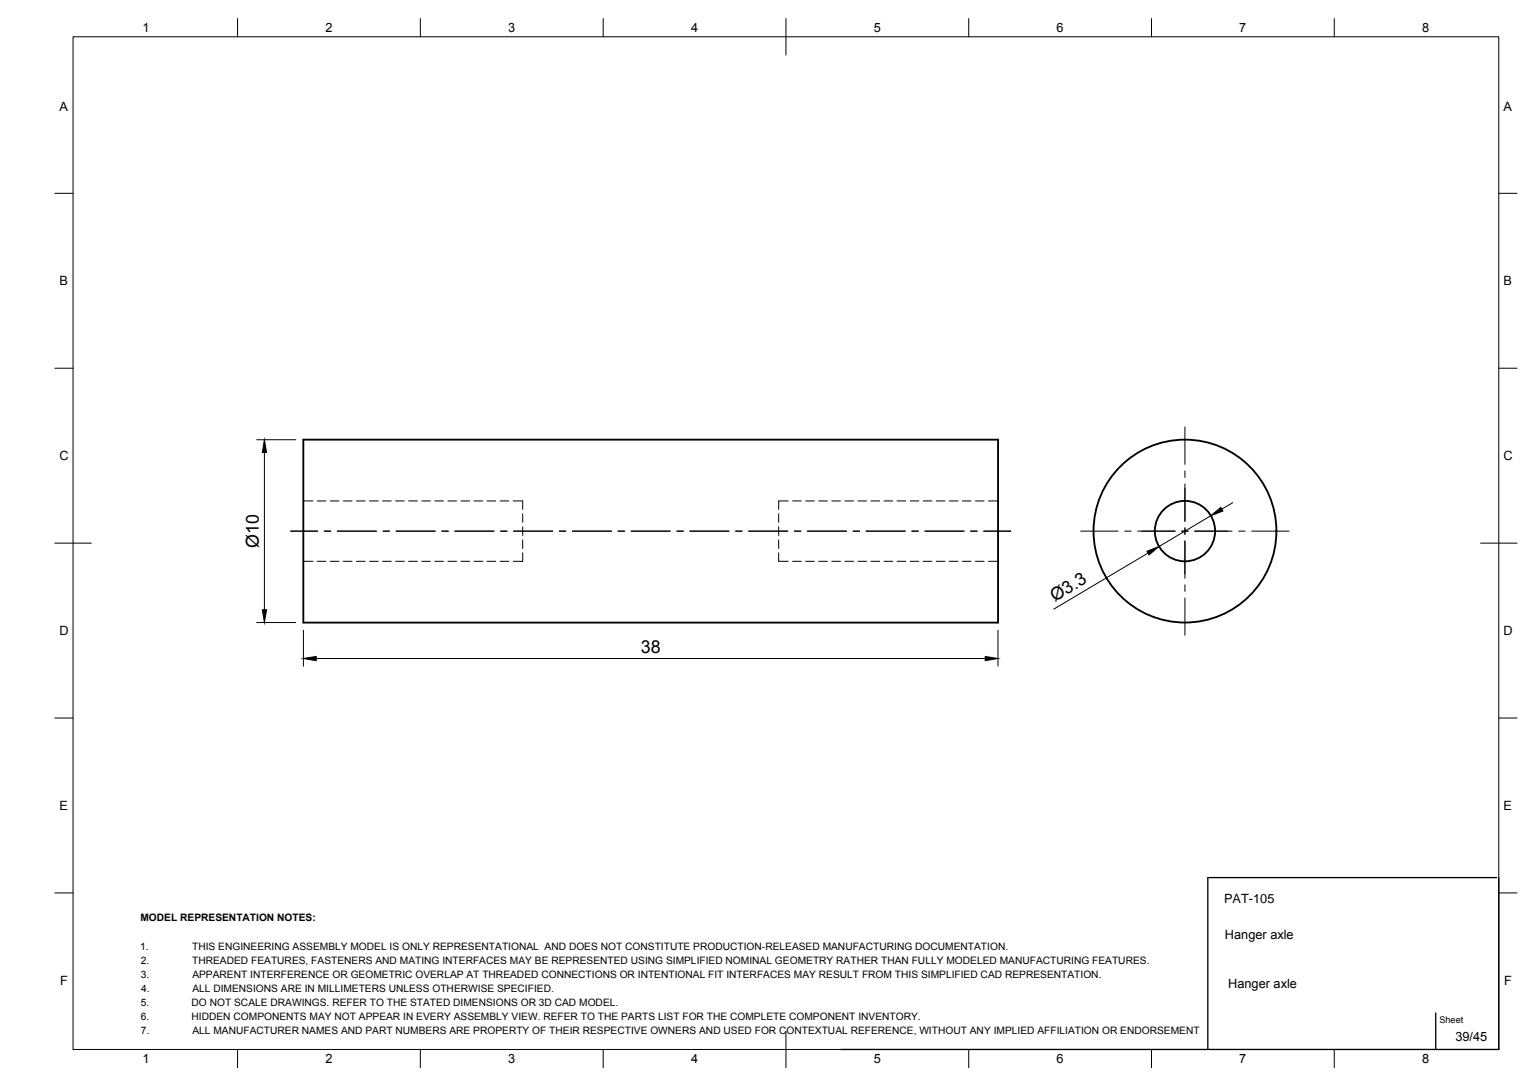
ISO-10303-21;
HEADER;
/* Generated by software containing ST-Developer
 * from STEP Tools, Inc. (www.steptools.com) 
 */

FILE_DESCRIPTION(
/* description */ ('Torque wrench calibration arm'),
/* implementation_level */ '2;1');

FILE_NAME(
/* name */ 'Hanger axle.step',
/* time_stamp */ '2026-10-28T03:24:52-07:00',
/* author */ (''),
/* organization */ (''),
/* preprocessor_version */ 'ST-DEVELOPER v20.2',
/* originating_system */ 'Autodesk Translation Framework v15.17.0.0',
/* authorisation */ '');

FILE_SCHEMA (('AUTOMOTIVE_DESIGN { 1 0 10303 214 3 1 1 }'));
ENDSEC;

DATA;
#10=MECHANICAL_DESIGN_GEOMETRIC_PRESENTATION_REPRESENTATION('',(#472),#12783);
#381=SHAPE_REPRESENTATION_RELATIONSHIP('SRR','None',#12966,#418);
#418=ADVANCED_BREP_SHAPE_REPRESENTATION('',(#524),#12775);
#472=STYLED_ITEM('',(#13212),#524);
#524=MANIFOLD_SOLID_BREP('Body1',#6543);
#637=FACE_BOUND('',#1730,.T.);
#638=FACE_BOUND('',#1732,.T.);
#848=PLANE('',#7709);
#849=PLANE('',#7713);
#850=PLANE('',#7717);
#851=PLANE('',#7718);
#1223=FACE_OUTER_BOUND('',#1724,.T.);
#1224=FACE_OUTER_BOUND('',#1725,.T.);
#1225=FACE_OUTER_BOUND('',#1726,.T.);
#1226=FACE_OUTER_BOUND('',#1727,.T.);
#1227=FACE_OUTER_BOUND('',#1728,.T.);
#1228=FACE_OUTER_BOUND('',#1729,.T.);
#1229=FACE_OUTER_BOUND('',#1731,.T.);
#1724=EDGE_LOOP('',(#5837,#5838,#5839,#5840));
#1725=EDGE_LOOP('',(#5841));
#1726=EDGE_LOOP('',(#5842,#5843,#5844,#5845));
#1727=EDGE_LOOP('',(#5846));
#1728=EDGE_LOOP('',(#5847,#5848,#5849,#5850));
#1729=EDGE_LOOP('',(#5851));
#1730=EDGE_LOOP('',(#5852));
#1731=EDGE_LOOP('',(#5853));
#1732=EDGE_LOOP('',(#5854));
#2163=LINE('',#12509,#2578);
#2164=LINE('',#12516,#2579);
#2165=LINE('',#12523,#2580);
#2578=VECTOR('',#9683,0.164999999999999);
#2579=VECTOR('',#9692,0.164999999999999);
#2580=VECTOR('',#9701,0.5);
#2934=CIRCLE('',#7707,0.164999999999999);
#2935=CIRCLE('',#7708,0.164999999999999);
#2936=CIRCLE('',#7711,0.164999999999999);
#2937=CIRCLE('',#7712,0.164999999999999);
#2938=CIRCLE('',#7715,0.5);
#2939=CIRCLE('',#7716,0.5);
#3484=VERTEX_POINT('',#12506);
#3485=VERTEX_POINT('',#12508);
#3486=VERTEX_POINT('',#12513);
#3487=VERTEX_POINT('',#12515);
#3488=VERTEX_POINT('',#12520);
#3489=VERTEX_POINT('',#12522);
#4276=EDGE_CURVE('',#3484,#3484,#2934,.T.);
#4277=EDGE_CURVE('',#3484,#3485,#2163,.T.);
#4278=EDGE_CURVE('',#3485,#3485,#2935,.T.);
#4279=EDGE_CURVE('',#3486,#3486,#2936,.T.);
#4280=EDGE_CURVE('',#3486,#3487,#2164,.T.);
#4281=EDGE_CURVE('',#3487,#3487,#2937,.T.);
#4282=EDGE_CURVE('',#3488,#3488,#2938,.T.);
#4283=EDGE_CURVE('',#3488,#3489,#2165,.T.);
#4284=EDGE_CURVE('',#3489,#3489,#2939,.T.);
#5837=ORIENTED_EDGE('',*,*,#4276,.F.);
#5838=ORIENTED_EDGE('',*,*,#4277,.T.);
#5839=ORIENTED_EDGE('',*,*,#4278,.F.);
#5840=ORIENTED_EDGE('',*,*,#4277,.F.);
#5841=ORIENTED_EDGE('',*,*,#4276,.T.);
#5842=ORIENTED_EDGE('',*,*,#4279,.F.);
#5843=ORIENTED_EDGE('',*,*,#4280,.T.);
#5844=ORIENTED_EDGE('',*,*,#4281,.T.);
#5845=ORIENTED_EDGE('',*,*,#4280,.F.);
#5846=ORIENTED_EDGE('',*,*,#4281,.F.);
#5847=ORIENTED_EDGE('',*,*,#4282,.F.);
#5848=ORIENTED_EDGE('',*,*,#4283,.T.);
#5849=ORIENTED_EDGE('',*,*,#4284,.T.);
#5850=ORIENTED_EDGE('',*,*,#4283,.F.);
#5851=ORIENTED_EDGE('',*,*,#4282,.T.);
#5852=ORIENTED_EDGE('',*,*,#4278,.T.);
#5853=ORIENTED_EDGE('',*,*,#4284,.F.);
#5854=ORIENTED_EDGE('',*,*,#4279,.T.);
#6083=CYLINDRICAL_SURFACE('',#7706,0.164999999999999);
#6084=CYLINDRICAL_SURFACE('',#7710,0.164999999999999);
#6085=CYLINDRICAL_SURFACE('',#7714,0.5);
#6448=ADVANCED_FACE('',(#1223),#6083,.F.);
#6449=ADVANCED_FACE('',(#1224),#848,.T.);
#6450=ADVANCED_FACE('',(#1225),#6084,.F.);
#6451=ADVANCED_FACE('',(#1226),#849,.F.);
#6452=ADVANCED_FACE('',(#1227),#6085,.T.);
#6453=ADVANCED_FACE('',(#1228,#637),#850,.T.);
#6454=ADVANCED_FACE('',(#1229,#638),#851,.F.);
#6543=CLOSED_SHELL('',(#6448,#6449,#6450,#6451,#6452,#6453,#6454));
#7705=AXIS2_PLACEMENT_3D('',#12504,#9677,#9678);
#7706=AXIS2_PLACEMENT_3D('',#12505,#9679,#9680);
#7707=AXIS2_PLACEMENT_3D('',#12507,#9681,#9682);
#7708=AXIS2_PLACEMENT_3D('',#12510,#9684,#9685);
#7709=AXIS2_PLACEMENT_3D('',#12511,#9686,#9687);
#7710=AXIS2_PLACEMENT_3D('',#12512,#9688,#9689);
#7711=AXIS2_PLACEMENT_3D('',#12514,#9690,#9691);
#7712=AXIS2_PLACEMENT_3D('',#12517,#9693,#9694);
#7713=AXIS2_PLACEMENT_3D('',#12518,#9695,#9696);
#7714=AXIS2_PLACEMENT_3D('',#12519,#9697,#9698);
#7715=AXIS2_PLACEMENT_3D('',#12521,#9699,#9700);
#7716=AXIS2_PLACEMENT_3D('',#12524,#9702,#9703);
#7717=AXIS2_PLACEMENT_3D('',#12525,#9704,#9705);
#7718=AXIS2_PLACEMENT_3D('',#12526,#9706,#9707);
#9677=DIRECTION('axis',(0.,0.,1.));
#9678=DIRECTION('refdir',(1.,0.,0.));
#9679=DIRECTION('center_axis',(0.,1.,0.));
#9680=DIRECTION('ref_axis',(1.,0.,0.));
#9681=DIRECTION('center_axis',(0.,1.,0.));
#9682=DIRECTION('ref_axis',(1.,0.,0.));
#9683=DIRECTION('',(0.,1.,0.));
#9684=DIRECTION('center_axis',(0.,-1.,0.));
#9685=DIRECTION('ref_axis',(1.,0.,0.));
#9686=DIRECTION('center_axis',(0.,1.,0.));
#9687=DIRECTION('ref_axis',(1.,0.,0.));
#9688=DIRECTION('center_axis',(0.,1.,0.));
#9689=DIRECTION('ref_axis',(1.,0.,0.));
#9690=DIRECTION('center_axis',(0.,1.,0.));
#9691=DIRECTION('ref_axis',(1.,0.,0.));
#9692=DIRECTION('',(0.,1.,0.));
#9693=DIRECTION('center_axis',(0.,1.,0.));
#9694=DIRECTION('ref_axis',(1.,0.,0.));
#9695=DIRECTION('center_axis',(0.,1.,0.));
#9696=DIRECTION('ref_axis',(1.,0.,0.));
#9697=DIRECTION('center_axis',(0.,1.,0.));
#9698=DIRECTION('ref_axis',(1.,0.,0.));
#9699=DIRECTION('center_axis',(0.,1.,0.));
#9700=DIRECTION('ref_axis',(1.,0.,0.));
#9701=DIRECTION('',(0.,-1.,0.));
#9702=DIRECTION('center_axis',(0.,1.,0.));
#9703=DIRECTION('ref_axis',(1.,0.,0.));
#9704=DIRECTION('center_axis',(0.,1.,0.));
#9705=DIRECTION('ref_axis',(1.,0.,0.));
#9706=DIRECTION('center_axis',(0.,1.,0.));
#9707=DIRECTION('ref_axis',(1.,0.,0.));
#12504=CARTESIAN_POINT('',(0.,0.,0.));
#12505=CARTESIAN_POINT('Origin',(50.,9.2,8.));
#12506=CARTESIAN_POINT('',(49.835,9.2,8.));
#12507=CARTESIAN_POINT('Origin',(50.,9.2,8.));
#12508=CARTESIAN_POINT('',(49.835,10.4,8.));
#12509=CARTESIAN_POINT('',(49.835,9.2,8.));
#12510=CARTESIAN_POINT('Origin',(50.,10.4,8.));
#12511=CARTESIAN_POINT('Origin',(50.,9.2,8.));
#12512=CARTESIAN_POINT('Origin',(50.,6.5,8.));
#12513=CARTESIAN_POINT('',(49.835,6.6,8.));
#12514=CARTESIAN_POINT('Origin',(50.,6.6,8.));
#12515=CARTESIAN_POINT('',(49.835,7.8,8.));
#12516=CARTESIAN_POINT('',(49.835,6.5,8.));
#12517=CARTESIAN_POINT('Origin',(50.,7.8,8.));
#12518=CARTESIAN_POINT('Origin',(50.,7.8,8.));
#12519=CARTESIAN_POINT('Origin',(50.,6.6,8.));
#12520=CARTESIAN_POINT('',(49.5,10.4,8.));
#12521=CARTESIAN_POINT('Origin',(50.,10.4,8.));
#12522=CARTESIAN_POINT('',(49.5,6.6,8.));
#12523=CARTESIAN_POINT('',(49.5,6.6,8.));
#12524=CARTESIAN_POINT('Origin',(50.,6.6,8.));
#12525=CARTESIAN_POINT('Origin',(50.,10.4,8.));
#12526=CARTESIAN_POINT('Origin',(50.,6.6,8.));
#12731=UNCERTAINTY_MEASURE_WITH_UNIT(LENGTH_MEASURE(0.001),#12784,
'DISTANCE_ACCURACY_VALUE',
'Maximum model space distance between geometric entities at asserted c
onnectivities');
#12739=UNCERTAINTY_MEASURE_WITH_UNIT(LENGTH_MEASURE(0.001),#12784,
'DISTANCE_ACCURACY_VALUE',
'Maximum model space distance between geometric entities at asserted c
onnectivities');
#12775=(
GEOMETRIC_REPRESENTATION_CONTEXT(3)
GLOBAL_UNCERTAINTY_ASSIGNED_CONTEXT((#12731))
GLOBAL_UNIT_ASSIGNED_CONTEXT((#12784,#12786,#12787))
REPRESENTATION_CONTEXT('','3D')
);
#12783=(
GEOMETRIC_REPRESENTATION_CONTEXT(3)
GLOBAL_UNCERTAINTY_ASSIGNED_CONTEXT((#12739))
GLOBAL_UNIT_ASSIGNED_CONTEXT((#12784,#12786,#12787))
REPRESENTATION_CONTEXT('','3D')
);
#12784=(
LENGTH_UNIT()
NAMED_UNIT(*)
SI_UNIT(.CENTI.,.METRE.)
);
#12786=(
NAMED_UNIT(*)
PLANE_ANGLE_UNIT()
SI_UNIT($,.RADIAN.)
);
#12787=(
NAMED_UNIT(*)
SI_UNIT($,.STERADIAN.)
SOLID_ANGLE_UNIT()
);
#12823=SHAPE_DEFINITION_REPRESENTATION(#12910,#12966);
#12910=PRODUCT_DEFINITION_SHAPE('',$,#13010);
#12966=SHAPE_REPRESENTATION('',(#7705),#12775);
#12974=PRODUCT_DEFINITION_CONTEXT('part definition',#13105,'design');
#13010=PRODUCT_DEFINITION('Hanger axle','Hanger axle',#13053,#12974);
#13053=PRODUCT_DEFINITION_FORMATION('',$,#13142);
#13105=APPLICATION_CONTEXT(
'Core Data for Automotive Mechanical Design Process');
#13106=PRODUCT_CONTEXT('part definition',#13105,'mechanical');
#13142=PRODUCT('Hanger axle','Hanger axle','Hanger axle',(#13106));
#13206=COLOUR_RGB('Grey',0.48,0.52,0.57);
#13207=FILL_AREA_STYLE_COLOUR('',#13206);
#13208=FILL_AREA_STYLE('',(#13207));
#13209=SURFACE_STYLE_FILL_AREA(#13208);
#13210=SURFACE_SIDE_STYLE('',(#13209));
#13211=SURFACE_STYLE_USAGE(.BOTH.,#13210);
#13212=PRESENTATION_STYLE_ASSIGNMENT((#13211));
ENDSEC;
END-ISO-10303-21;
